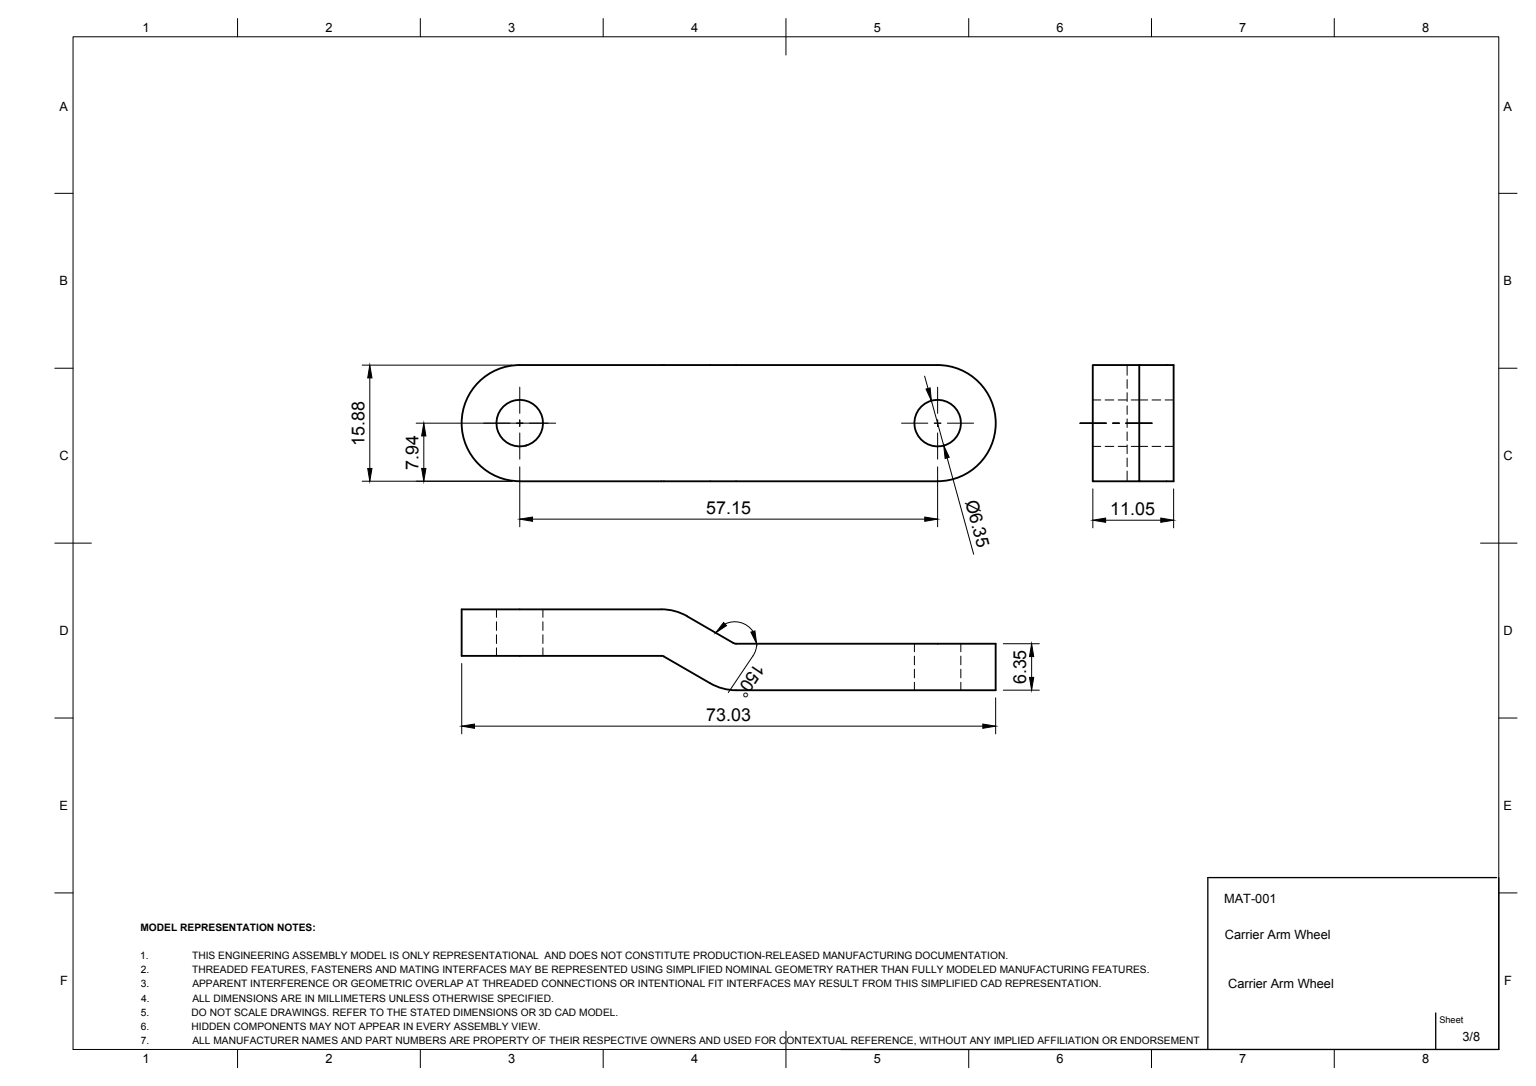
ISO-10303-21;
HEADER;
/* Generated by software containing ST-Developer
 * from STEP Tools, Inc. (www.steptools.com) 
 */

FILE_DESCRIPTION(
/* description */ ('STEP AP214'),
/* implementation_level */ '2;1');

FILE_NAME(
/* name */ 'Carrier Arm Wheel.step',
/* time_stamp */ '2026-11-14T04:30:00-08:00',
/* author */ (''),
/* organization */ (''),
/* preprocessor_version */ 'ST-DEVELOPER v20.2',
/* originating_system */ 'Autodesk Translation Framework v15.17.0.0',
/* authorisation */ '');

FILE_SCHEMA (('AUTOMOTIVE_DESIGN { 1 0 10303 214 3 1 1 }'));
ENDSEC;

DATA;
#10=MECHANICAL_DESIGN_GEOMETRIC_PRESENTATION_REPRESENTATION('',(#129),#40809);
#113=SHAPE_REPRESENTATION_RELATIONSHIP('SRR','None',#40863,#121);
#121=ADVANCED_BREP_SHAPE_REPRESENTATION('',(#137),#40807);
#129=STYLED_ITEM('',(#40906),#137);
#137=MANIFOLD_SOLID_BREP('Body1',#6304);
#313=PLANE('',#7024);
#314=PLANE('',#7025);
#315=PLANE('',#7026);
#316=PLANE('',#7027);
#317=PLANE('',#7031);
#318=PLANE('',#7032);
#319=PLANE('',#7033);
#320=PLANE('',#7034);
#321=PLANE('',#7035);
#322=PLANE('',#7038);
#323=PLANE('',#7043);
#324=PLANE('',#7046);
#325=PLANE('',#7051);
#326=PLANE('',#7052);
#327=PLANE('',#7053);
#328=PLANE('',#7054);
#355=FACE_BOUND('',#1227,.T.);
#356=FACE_BOUND('',#1230,.T.);
#357=FACE_BOUND('',#1241,.T.);
#358=FACE_BOUND('',#1244,.T.);
#815=FACE_OUTER_BOUND('',#1218,.T.);
#816=FACE_OUTER_BOUND('',#1219,.T.);
#817=FACE_OUTER_BOUND('',#1220,.T.);
#818=FACE_OUTER_BOUND('',#1221,.T.);
#819=FACE_OUTER_BOUND('',#1222,.T.);
#820=FACE_OUTER_BOUND('',#1223,.T.);
#821=FACE_OUTER_BOUND('',#1224,.T.);
#822=FACE_OUTER_BOUND('',#1225,.T.);
#823=FACE_OUTER_BOUND('',#1226,.T.);
#824=FACE_OUTER_BOUND('',#1228,.T.);
#825=FACE_OUTER_BOUND('',#1229,.T.);
#826=FACE_OUTER_BOUND('',#1231,.T.);
#827=FACE_OUTER_BOUND('',#1232,.T.);
#828=FACE_OUTER_BOUND('',#1233,.T.);
#829=FACE_OUTER_BOUND('',#1234,.T.);
#830=FACE_OUTER_BOUND('',#1235,.T.);
#831=FACE_OUTER_BOUND('',#1236,.T.);
#832=FACE_OUTER_BOUND('',#1237,.T.);
#833=FACE_OUTER_BOUND('',#1238,.T.);
#834=FACE_OUTER_BOUND('',#1239,.T.);
#835=FACE_OUTER_BOUND('',#1240,.T.);
#836=FACE_OUTER_BOUND('',#1242,.T.);
#837=FACE_OUTER_BOUND('',#1243,.T.);
#838=FACE_OUTER_BOUND('',#1245,.T.);
#1218=EDGE_LOOP('',(#5478,#5479,#5480,#5481));
#1219=EDGE_LOOP('',(#5482,#5483,#5484,#5485));
#1220=EDGE_LOOP('',(#5486,#5487,#5488,#5489));
#1221=EDGE_LOOP('',(#5490,#5491,#5492,#5493));
#1222=EDGE_LOOP('',(#5494,#5495,#5496,#5497));
#1223=EDGE_LOOP('',(#5498,#5499,#5500,#5501));
#1224=EDGE_LOOP('',(#5502,#5503,#5504,#5505));
#1225=EDGE_LOOP('',(#5506,#5507,#5508,#5509));
#1226=EDGE_LOOP('',(#5510,#5511,#5512,#5513));
#1227=EDGE_LOOP('',(#5514));
#1228=EDGE_LOOP('',(#5515,#5516,#5517,#5518));
#1229=EDGE_LOOP('',(#5519,#5520,#5521,#5522));
#1230=EDGE_LOOP('',(#5523));
#1231=EDGE_LOOP('',(#5524,#5525,#5526,#5527));
#1232=EDGE_LOOP('',(#5528,#5529,#5530,#5531));
#1233=EDGE_LOOP('',(#5532,#5533,#5534,#5535));
#1234=EDGE_LOOP('',(#5536,#5537,#5538,#5539));
#1235=EDGE_LOOP('',(#5540,#5541,#5542,#5543));
#1236=EDGE_LOOP('',(#5544,#5545,#5546,#5547));
#1237=EDGE_LOOP('',(#5548,#5549,#5550,#5551));
#1238=EDGE_LOOP('',(#5552,#5553,#5554,#5555));
#1239=EDGE_LOOP('',(#5556,#5557,#5558,#5559));
#1240=EDGE_LOOP('',(#5560,#5561,#5562,#5563));
#1241=EDGE_LOOP('',(#5564));
#1242=EDGE_LOOP('',(#5565,#5566,#5567,#5568));
#1243=EDGE_LOOP('',(#5569,#5570,#5571,#5572));
#1244=EDGE_LOOP('',(#5573));
#1245=EDGE_LOOP('',(#5574,#5575,#5576,#5577));
#1623=CIRCLE('',#7016,3.175);
#1624=CIRCLE('',#7017,3.175);
#1625=CIRCLE('',#7019,7.94000000000001);
#1626=CIRCLE('',#7020,7.94000000000001);
#1627=CIRCLE('',#7022,3.175);
#1628=CIRCLE('',#7023,3.175);
#1629=CIRCLE('',#7029,7.94000000000001);
#1630=CIRCLE('',#7030,7.94000000000001);
#1631=CIRCLE('',#7036,0.7366);
#1632=CIRCLE('',#7037,7.0866);
#1633=CIRCLE('',#7039,0.7366);
#1634=CIRCLE('',#7040,7.0866);
#1635=CIRCLE('',#7044,7.0866);
#1636=CIRCLE('',#7045,0.7366);
#1637=CIRCLE('',#7047,7.0866);
#1638=CIRCLE('',#7048,0.7366);
#2071=LINE('',#40433,#2389);
#2072=LINE('',#40440,#2390);
#2073=LINE('',#40443,#2391);
#2074=LINE('',#40448,#2392);
#2075=LINE('',#40453,#2393);
#2076=LINE('',#40455,#2394);
#2077=LINE('',#40457,#2395);
#2078=LINE('',#40458,#2396);
#2079=LINE('',#40462,#2397);
#2080=LINE('',#40463,#2398);
#2081=LINE('',#40464,#2399);
#2082=LINE('',#40467,#2400);
#2083=LINE('',#40469,#2401);
#2084=LINE('',#40470,#2402);
#2085=LINE('',#40472,#2403);
#2086=LINE('',#40473,#2404);
#2087=LINE('',#40479,#2405);
#2088=LINE('',#40482,#2406);
#2089=LINE('',#40486,#2407);
#2090=LINE('',#40487,#2408);
#2091=LINE('',#40488,#2409);
#2092=LINE('',#40491,#2410);
#2093=LINE('',#40492,#2411);
#2094=LINE('',#40495,#2412);
#2095=LINE('',#40496,#2413);
#2096=LINE('',#40498,#2414);
#2097=LINE('',#40510,#2415);
#2098=LINE('',#40517,#2416);
#2099=LINE('',#40520,#2417);
#2100=LINE('',#40522,#2418);
#2101=LINE('',#40524,#2419);
#2102=LINE('',#40525,#2420);
#2103=LINE('',#40527,#2421);
#2104=LINE('',#40529,#2422);
#2389=VECTOR('',#8673,3.175);
#2390=VECTOR('',#8680,1000.);
#2391=VECTOR('',#8683,1000.);
#2392=VECTOR('',#8688,3.175);
#2393=VECTOR('',#8693,1000.);
#2394=VECTOR('',#8694,1000.);
#2395=VECTOR('',#8695,1000.);
#2396=VECTOR('',#8696,1000.);
#2397=VECTOR('',#8699,1000.);
#2398=VECTOR('',#8700,1000.);
#2399=VECTOR('',#8701,1000.);
#2400=VECTOR('',#8704,1000.);
#2401=VECTOR('',#8705,1000.);
#2402=VECTOR('',#8706,1000.);
#2403=VECTOR('',#8709,1000.);
#2404=VECTOR('',#8710,1000.);
#2405=VECTOR('',#8715,1000.);
#2406=VECTOR('',#8718,1000.);
#2407=VECTOR('',#8721,1000.);
#2408=VECTOR('',#8722,1000.);
#2409=VECTOR('',#8723,1000.);
#2410=VECTOR('',#8726,1000.);
#2411=VECTOR('',#8727,1000.);
#2412=VECTOR('',#8730,1000.);
#2413=VECTOR('',#8731,1000.);
#2414=VECTOR('',#8734,1000.);
#2415=VECTOR('',#8753,1000.);
#2416=VECTOR('',#8762,1000.);
#2417=VECTOR('',#8767,1000.);
#2418=VECTOR('',#8770,1000.);
#2419=VECTOR('',#8773,1000.);
#2420=VECTOR('',#8774,1000.);
#2421=VECTOR('',#8777,1000.);
#2422=VECTOR('',#8780,1000.);
#2935=VERTEX_POINT('',#40430);
#2936=VERTEX_POINT('',#40432);
#2937=VERTEX_POINT('',#40436);
#2938=VERTEX_POINT('',#40437);
#2939=VERTEX_POINT('',#40439);
#2940=VERTEX_POINT('',#40441);
#2941=VERTEX_POINT('',#40445);
#2942=VERTEX_POINT('',#40447);
#2943=VERTEX_POINT('',#40451);
#2944=VERTEX_POINT('',#40452);
#2945=VERTEX_POINT('',#40454);
#2946=VERTEX_POINT('',#40456);
#2947=VERTEX_POINT('',#40460);
#2948=VERTEX_POINT('',#40461);
#2949=VERTEX_POINT('',#40466);
#2950=VERTEX_POINT('',#40468);
#2951=VERTEX_POINT('',#40475);
#2952=VERTEX_POINT('',#40476);
#2953=VERTEX_POINT('',#40478);
#2954=VERTEX_POINT('',#40480);
#2955=VERTEX_POINT('',#40484);
#2956=VERTEX_POINT('',#40485);
#2957=VERTEX_POINT('',#40490);
#2958=VERTEX_POINT('',#40494);
#2959=VERTEX_POINT('',#40508);
#2960=VERTEX_POINT('',#40509);
#2961=VERTEX_POINT('',#40514);
#2962=VERTEX_POINT('',#40516);
#3791=EDGE_CURVE('',#2935,#2935,#1623,.T.);
#3792=EDGE_CURVE('',#2935,#2936,#2071,.T.);
#3793=EDGE_CURVE('',#2936,#2936,#1624,.T.);
#3794=EDGE_CURVE('',#2937,#2938,#1625,.T.);
#3795=EDGE_CURVE('',#2938,#2939,#2072,.T.);
#3796=EDGE_CURVE('',#2940,#2939,#1626,.T.);
#3797=EDGE_CURVE('',#2937,#2940,#2073,.T.);
#3798=EDGE_CURVE('',#2941,#2941,#1627,.T.);
#3799=EDGE_CURVE('',#2941,#2942,#2074,.T.);
#3800=EDGE_CURVE('',#2942,#2942,#1628,.T.);
#3801=EDGE_CURVE('',#2943,#2944,#2075,.T.);
#3802=EDGE_CURVE('',#2944,#2945,#2076,.T.);
#3803=EDGE_CURVE('',#2945,#2946,#2077,.T.);
#3804=EDGE_CURVE('',#2943,#2946,#2078,.T.);
#3805=EDGE_CURVE('',#2947,#2948,#2079,.T.);
#3806=EDGE_CURVE('',#2948,#2944,#2080,.T.);
#3807=EDGE_CURVE('',#2947,#2943,#2081,.T.);
#3808=EDGE_CURVE('',#2945,#2949,#2082,.T.);
#3809=EDGE_CURVE('',#2949,#2950,#2083,.T.);
#3810=EDGE_CURVE('',#2946,#2950,#2084,.T.);
#3811=EDGE_CURVE('',#2948,#2949,#2085,.T.);
#3812=EDGE_CURVE('',#2947,#2950,#2086,.T.);
#3813=EDGE_CURVE('',#2951,#2952,#1629,.T.);
#3814=EDGE_CURVE('',#2953,#2951,#2087,.T.);
#3815=EDGE_CURVE('',#2953,#2954,#1630,.T.);
#3816=EDGE_CURVE('',#2954,#2952,#2088,.T.);
#3817=EDGE_CURVE('',#2955,#2956,#2089,.T.);
#3818=EDGE_CURVE('',#2954,#2955,#2090,.T.);
#3819=EDGE_CURVE('',#2956,#2953,#2091,.T.);
#3820=EDGE_CURVE('',#2955,#2957,#2092,.T.);
#3821=EDGE_CURVE('',#2952,#2957,#2093,.T.);
#3822=EDGE_CURVE('',#2957,#2958,#2094,.T.);
#3823=EDGE_CURVE('',#2958,#2951,#2095,.T.);
#3824=EDGE_CURVE('',#2958,#2956,#2096,.T.);
#3825=EDGE_CURVE('',#2943,#2957,#1631,.T.);
#3826=EDGE_CURVE('',#2947,#2955,#1632,.T.);
#3827=EDGE_CURVE('',#2958,#2946,#1633,.T.);
#3828=EDGE_CURVE('',#2956,#2950,#1634,.T.);
#3829=EDGE_CURVE('',#2959,#2960,#2097,.T.);
#3830=EDGE_CURVE('',#2960,#2944,#1635,.T.);
#3831=EDGE_CURVE('',#2959,#2948,#1636,.T.);
#3832=EDGE_CURVE('',#2945,#2961,#1637,.T.);
#3833=EDGE_CURVE('',#2961,#2962,#2098,.T.);
#3834=EDGE_CURVE('',#2949,#2962,#1638,.T.);
#3835=EDGE_CURVE('',#2959,#2962,#2099,.T.);
#3836=EDGE_CURVE('',#2960,#2961,#2100,.T.);
#3837=EDGE_CURVE('',#2959,#2937,#2101,.T.);
#3838=EDGE_CURVE('',#2938,#2962,#2102,.T.);
#3839=EDGE_CURVE('',#2939,#2961,#2103,.T.);
#3840=EDGE_CURVE('',#2960,#2940,#2104,.T.);
#5478=ORIENTED_EDGE('',*,*,#3791,.F.);
#5479=ORIENTED_EDGE('',*,*,#3792,.T.);
#5480=ORIENTED_EDGE('',*,*,#3793,.T.);
#5481=ORIENTED_EDGE('',*,*,#3792,.F.);
#5482=ORIENTED_EDGE('',*,*,#3794,.T.);
#5483=ORIENTED_EDGE('',*,*,#3795,.T.);
#5484=ORIENTED_EDGE('',*,*,#3796,.F.);
#5485=ORIENTED_EDGE('',*,*,#3797,.F.);
#5486=ORIENTED_EDGE('',*,*,#3798,.F.);
#5487=ORIENTED_EDGE('',*,*,#3799,.T.);
#5488=ORIENTED_EDGE('',*,*,#3800,.T.);
#5489=ORIENTED_EDGE('',*,*,#3799,.F.);
#5490=ORIENTED_EDGE('',*,*,#3801,.T.);
#5491=ORIENTED_EDGE('',*,*,#3802,.T.);
#5492=ORIENTED_EDGE('',*,*,#3803,.T.);
#5493=ORIENTED_EDGE('',*,*,#3804,.F.);
#5494=ORIENTED_EDGE('',*,*,#3805,.T.);
#5495=ORIENTED_EDGE('',*,*,#3806,.T.);
#5496=ORIENTED_EDGE('',*,*,#3801,.F.);
#5497=ORIENTED_EDGE('',*,*,#3807,.F.);
#5498=ORIENTED_EDGE('',*,*,#3803,.F.);
#5499=ORIENTED_EDGE('',*,*,#3808,.T.);
#5500=ORIENTED_EDGE('',*,*,#3809,.T.);
#5501=ORIENTED_EDGE('',*,*,#3810,.F.);
#5502=ORIENTED_EDGE('',*,*,#3811,.F.);
#5503=ORIENTED_EDGE('',*,*,#3805,.F.);
#5504=ORIENTED_EDGE('',*,*,#3812,.T.);
#5505=ORIENTED_EDGE('',*,*,#3809,.F.);
#5506=ORIENTED_EDGE('',*,*,#3813,.F.);
#5507=ORIENTED_EDGE('',*,*,#3814,.F.);
#5508=ORIENTED_EDGE('',*,*,#3815,.T.);
#5509=ORIENTED_EDGE('',*,*,#3816,.T.);
#5510=ORIENTED_EDGE('',*,*,#3817,.F.);
#5511=ORIENTED_EDGE('',*,*,#3818,.F.);
#5512=ORIENTED_EDGE('',*,*,#3815,.F.);
#5513=ORIENTED_EDGE('',*,*,#3819,.F.);
#5514=ORIENTED_EDGE('',*,*,#3798,.T.);
#5515=ORIENTED_EDGE('',*,*,#3818,.T.);
#5516=ORIENTED_EDGE('',*,*,#3820,.T.);
#5517=ORIENTED_EDGE('',*,*,#3821,.F.);
#5518=ORIENTED_EDGE('',*,*,#3816,.F.);
#5519=ORIENTED_EDGE('',*,*,#3821,.T.);
#5520=ORIENTED_EDGE('',*,*,#3822,.T.);
#5521=ORIENTED_EDGE('',*,*,#3823,.T.);
#5522=ORIENTED_EDGE('',*,*,#3813,.T.);
#5523=ORIENTED_EDGE('',*,*,#3800,.F.);
#5524=ORIENTED_EDGE('',*,*,#3823,.F.);
#5525=ORIENTED_EDGE('',*,*,#3824,.T.);
#5526=ORIENTED_EDGE('',*,*,#3819,.T.);
#5527=ORIENTED_EDGE('',*,*,#3814,.T.);
#5528=ORIENTED_EDGE('',*,*,#3807,.T.);
#5529=ORIENTED_EDGE('',*,*,#3825,.T.);
#5530=ORIENTED_EDGE('',*,*,#3820,.F.);
#5531=ORIENTED_EDGE('',*,*,#3826,.F.);
#5532=ORIENTED_EDGE('',*,*,#3824,.F.);
#5533=ORIENTED_EDGE('',*,*,#3827,.T.);
#5534=ORIENTED_EDGE('',*,*,#3810,.T.);
#5535=ORIENTED_EDGE('',*,*,#3828,.F.);
#5536=ORIENTED_EDGE('',*,*,#3828,.T.);
#5537=ORIENTED_EDGE('',*,*,#3812,.F.);
#5538=ORIENTED_EDGE('',*,*,#3826,.T.);
#5539=ORIENTED_EDGE('',*,*,#3817,.T.);
#5540=ORIENTED_EDGE('',*,*,#3827,.F.);
#5541=ORIENTED_EDGE('',*,*,#3822,.F.);
#5542=ORIENTED_EDGE('',*,*,#3825,.F.);
#5543=ORIENTED_EDGE('',*,*,#3804,.T.);
#5544=ORIENTED_EDGE('',*,*,#3829,.T.);
#5545=ORIENTED_EDGE('',*,*,#3830,.T.);
#5546=ORIENTED_EDGE('',*,*,#3806,.F.);
#5547=ORIENTED_EDGE('',*,*,#3831,.F.);
#5548=ORIENTED_EDGE('',*,*,#3808,.F.);
#5549=ORIENTED_EDGE('',*,*,#3832,.T.);
#5550=ORIENTED_EDGE('',*,*,#3833,.T.);
#5551=ORIENTED_EDGE('',*,*,#3834,.F.);
#5552=ORIENTED_EDGE('',*,*,#3834,.T.);
#5553=ORIENTED_EDGE('',*,*,#3835,.F.);
#5554=ORIENTED_EDGE('',*,*,#3831,.T.);
#5555=ORIENTED_EDGE('',*,*,#3811,.T.);
#5556=ORIENTED_EDGE('',*,*,#3832,.F.);
#5557=ORIENTED_EDGE('',*,*,#3802,.F.);
#5558=ORIENTED_EDGE('',*,*,#3830,.F.);
#5559=ORIENTED_EDGE('',*,*,#3836,.T.);
#5560=ORIENTED_EDGE('',*,*,#3837,.F.);
#5561=ORIENTED_EDGE('',*,*,#3835,.T.);
#5562=ORIENTED_EDGE('',*,*,#3838,.F.);
#5563=ORIENTED_EDGE('',*,*,#3794,.F.);
#5564=ORIENTED_EDGE('',*,*,#3791,.T.);
#5565=ORIENTED_EDGE('',*,*,#3833,.F.);
#5566=ORIENTED_EDGE('',*,*,#3839,.F.);
#5567=ORIENTED_EDGE('',*,*,#3795,.F.);
#5568=ORIENTED_EDGE('',*,*,#3838,.T.);
#5569=ORIENTED_EDGE('',*,*,#3836,.F.);
#5570=ORIENTED_EDGE('',*,*,#3840,.T.);
#5571=ORIENTED_EDGE('',*,*,#3796,.T.);
#5572=ORIENTED_EDGE('',*,*,#3839,.T.);
#5573=ORIENTED_EDGE('',*,*,#3793,.F.);
#5574=ORIENTED_EDGE('',*,*,#3829,.F.);
#5575=ORIENTED_EDGE('',*,*,#3837,.T.);
#5576=ORIENTED_EDGE('',*,*,#3797,.T.);
#5577=ORIENTED_EDGE('',*,*,#3840,.F.);
#5889=CYLINDRICAL_SURFACE('',#7015,3.175);
#5890=CYLINDRICAL_SURFACE('',#7018,7.94000000000001);
#5891=CYLINDRICAL_SURFACE('',#7021,3.175);
#5892=CYLINDRICAL_SURFACE('',#7028,7.94000000000001);
#5893=CYLINDRICAL_SURFACE('',#7041,7.0866);
#5894=CYLINDRICAL_SURFACE('',#7042,0.7366);
#5895=CYLINDRICAL_SURFACE('',#7049,0.7366);
#5896=CYLINDRICAL_SURFACE('',#7050,7.0866);
#6230=ADVANCED_FACE('',(#815),#5889,.F.);
#6231=ADVANCED_FACE('',(#816),#5890,.T.);
#6232=ADVANCED_FACE('',(#817),#5891,.F.);
#6233=ADVANCED_FACE('',(#818),#313,.T.);
#6234=ADVANCED_FACE('',(#819),#314,.T.);
#6235=ADVANCED_FACE('',(#820),#315,.T.);
#6236=ADVANCED_FACE('',(#821),#316,.F.);
#6237=ADVANCED_FACE('',(#822),#5892,.T.);
#6238=ADVANCED_FACE('',(#823,#355),#317,.F.);
#6239=ADVANCED_FACE('',(#824),#318,.T.);
#6240=ADVANCED_FACE('',(#825,#356),#319,.T.);
#6241=ADVANCED_FACE('',(#826),#320,.T.);
#6242=ADVANCED_FACE('',(#827),#321,.T.);
#6243=ADVANCED_FACE('',(#828),#322,.T.);
#6244=ADVANCED_FACE('',(#829),#5893,.T.);
#6245=ADVANCED_FACE('',(#830),#5894,.F.);
#6246=ADVANCED_FACE('',(#831),#323,.F.);
#6247=ADVANCED_FACE('',(#832),#324,.F.);
#6248=ADVANCED_FACE('',(#833),#5895,.F.);
#6249=ADVANCED_FACE('',(#834),#5896,.T.);
#6250=ADVANCED_FACE('',(#835,#357),#325,.F.);
#6251=ADVANCED_FACE('',(#836),#326,.T.);
#6252=ADVANCED_FACE('',(#837,#358),#327,.T.);
#6253=ADVANCED_FACE('',(#838),#328,.T.);
#6304=CLOSED_SHELL('',(#6230,#6231,#6232,#6233,#6234,#6235,#6236,#6237,
#6238,#6239,#6240,#6241,#6242,#6243,#6244,#6245,#6246,#6247,#6248,#6249,
#6250,#6251,#6252,#6253));
#7014=AXIS2_PLACEMENT_3D('',#40428,#8667,#8668);
#7015=AXIS2_PLACEMENT_3D('',#40429,#8669,#8670);
#7016=AXIS2_PLACEMENT_3D('',#40431,#8671,#8672);
#7017=AXIS2_PLACEMENT_3D('',#40434,#8674,#8675);
#7018=AXIS2_PLACEMENT_3D('',#40435,#8676,#8677);
#7019=AXIS2_PLACEMENT_3D('',#40438,#8678,#8679);
#7020=AXIS2_PLACEMENT_3D('',#40442,#8681,#8682);
#7021=AXIS2_PLACEMENT_3D('',#40444,#8684,#8685);
#7022=AXIS2_PLACEMENT_3D('',#40446,#8686,#8687);
#7023=AXIS2_PLACEMENT_3D('',#40449,#8689,#8690);
#7024=AXIS2_PLACEMENT_3D('',#40450,#8691,#8692);
#7025=AXIS2_PLACEMENT_3D('',#40459,#8697,#8698);
#7026=AXIS2_PLACEMENT_3D('',#40465,#8702,#8703);
#7027=AXIS2_PLACEMENT_3D('',#40471,#8707,#8708);
#7028=AXIS2_PLACEMENT_3D('',#40474,#8711,#8712);
#7029=AXIS2_PLACEMENT_3D('',#40477,#8713,#8714);
#7030=AXIS2_PLACEMENT_3D('',#40481,#8716,#8717);
#7031=AXIS2_PLACEMENT_3D('',#40483,#8719,#8720);
#7032=AXIS2_PLACEMENT_3D('',#40489,#8724,#8725);
#7033=AXIS2_PLACEMENT_3D('',#40493,#8728,#8729);
#7034=AXIS2_PLACEMENT_3D('',#40497,#8732,#8733);
#7035=AXIS2_PLACEMENT_3D('',#40499,#8735,#8736);
#7036=AXIS2_PLACEMENT_3D('',#40500,#8737,#8738);
#7037=AXIS2_PLACEMENT_3D('',#40501,#8739,#8740);
#7038=AXIS2_PLACEMENT_3D('',#40502,#8741,#8742);
#7039=AXIS2_PLACEMENT_3D('',#40503,#8743,#8744);
#7040=AXIS2_PLACEMENT_3D('',#40504,#8745,#8746);
#7041=AXIS2_PLACEMENT_3D('',#40505,#8747,#8748);
#7042=AXIS2_PLACEMENT_3D('',#40506,#8749,#8750);
#7043=AXIS2_PLACEMENT_3D('',#40507,#8751,#8752);
#7044=AXIS2_PLACEMENT_3D('',#40511,#8754,#8755);
#7045=AXIS2_PLACEMENT_3D('',#40512,#8756,#8757);
#7046=AXIS2_PLACEMENT_3D('',#40513,#8758,#8759);
#7047=AXIS2_PLACEMENT_3D('',#40515,#8760,#8761);
#7048=AXIS2_PLACEMENT_3D('',#40518,#8763,#8764);
#7049=AXIS2_PLACEMENT_3D('',#40519,#8765,#8766);
#7050=AXIS2_PLACEMENT_3D('',#40521,#8768,#8769);
#7051=AXIS2_PLACEMENT_3D('',#40523,#8771,#8772);
#7052=AXIS2_PLACEMENT_3D('',#40526,#8775,#8776);
#7053=AXIS2_PLACEMENT_3D('',#40528,#8778,#8779);
#7054=AXIS2_PLACEMENT_3D('',#40530,#8781,#8782);
#8667=DIRECTION('axis',(0.,0.,1.));
#8668=DIRECTION('refdir',(1.,0.,0.));
#8669=DIRECTION('center_axis',(1.,0.,0.));
#8670=DIRECTION('ref_axis',(0.,0.,-1.));
#8671=DIRECTION('center_axis',(1.,0.,0.));
#8672=DIRECTION('ref_axis',(0.,0.,-1.));
#8673=DIRECTION('',(1.,0.,0.));
#8674=DIRECTION('center_axis',(1.,0.,0.));
#8675=DIRECTION('ref_axis',(0.,0.,-1.));
#8676=DIRECTION('center_axis',(1.,0.,0.));
#8677=DIRECTION('ref_axis',(0.,0.,-1.));
#8678=DIRECTION('center_axis',(1.,0.,0.));
#8679=DIRECTION('ref_axis',(0.,0.,-1.));
#8680=DIRECTION('',(1.,0.,0.));
#8681=DIRECTION('center_axis',(1.,0.,0.));
#8682=DIRECTION('ref_axis',(0.,0.,-1.));
#8683=DIRECTION('',(1.,0.,0.));
#8684=DIRECTION('center_axis',(1.,0.,0.));
#8685=DIRECTION('ref_axis',(0.,0.,-1.));
#8686=DIRECTION('center_axis',(1.,0.,0.));
#8687=DIRECTION('ref_axis',(0.,0.,-1.));
#8688=DIRECTION('',(1.,0.,0.));
#8689=DIRECTION('center_axis',(1.,0.,0.));
#8690=DIRECTION('ref_axis',(0.,0.,-1.));
#8691=DIRECTION('center_axis',(0.866025403784438,0.,0.500000000000001));
#8692=DIRECTION('ref_axis',(0.500000000000001,0.,-0.866025403784438));
#8693=DIRECTION('',(0.500000000000001,1.82123199577618E-16,-0.866025403784438));
#8694=DIRECTION('',(0.,1.,0.));
#8695=DIRECTION('',(-0.500000000000001,-1.82123199577618E-16,0.866025403784438));
#8696=DIRECTION('',(0.,1.,0.));
#8697=DIRECTION('center_axis',(9.10615997888089E-17,-1.,-1.5772331745272E-16));
#8698=DIRECTION('ref_axis',(0.500000000000001,1.82123199577618E-16,-0.866025403784438));
#8699=DIRECTION('',(0.500000000000001,1.82123199577618E-16,-0.866025403784438));
#8700=DIRECTION('',(0.866025403784438,1.11518296706602E-32,0.500000000000001));
#8701=DIRECTION('',(0.866025403784438,1.11518296706602E-32,0.500000000000001));
#8702=DIRECTION('center_axis',(-9.10615997888089E-17,1.,1.5772331745272E-16));
#8703=DIRECTION('ref_axis',(-0.500000000000001,-1.82123199577618E-16,0.866025403784438));
#8704=DIRECTION('',(-0.866025403784438,-1.11518296706602E-32,-0.500000000000001));
#8705=DIRECTION('',(-0.500000000000001,-1.82123199577618E-16,0.866025403784438));
#8706=DIRECTION('',(-0.866025403784438,-1.11518296706602E-32,-0.500000000000001));
#8707=DIRECTION('center_axis',(0.866025403784438,0.,0.500000000000001));
#8708=DIRECTION('ref_axis',(0.500000000000001,0.,-0.866025403784438));
#8709=DIRECTION('',(0.,1.,0.));
#8710=DIRECTION('',(0.,1.,0.));
#8711=DIRECTION('center_axis',(1.,0.,0.));
#8712=DIRECTION('ref_axis',(0.,1.22464679914735E-16,1.));
#8713=DIRECTION('center_axis',(1.,0.,0.));
#8714=DIRECTION('ref_axis',(0.,0.,-1.));
#8715=DIRECTION('',(1.,0.,0.));
#8716=DIRECTION('center_axis',(1.,0.,0.));
#8717=DIRECTION('ref_axis',(0.,0.,-1.));
#8718=DIRECTION('',(1.,0.,0.));
#8719=DIRECTION('center_axis',(1.,0.,0.));
#8720=DIRECTION('ref_axis',(0.,0.,-1.));
#8721=DIRECTION('',(0.,1.,0.));
#8722=DIRECTION('',(0.,1.82123199577618E-16,-1.));
#8723=DIRECTION('',(0.,-1.82123199577618E-16,1.));
#8724=DIRECTION('center_axis',(0.,-1.,-1.82123199577617E-16));
#8725=DIRECTION('ref_axis',(0.,1.82123199577618E-16,-1.));
#8726=DIRECTION('',(1.,1.11518296706602E-32,-6.12323399573677E-17));
#8727=DIRECTION('',(0.,1.82123199577618E-16,-1.));
#8728=DIRECTION('center_axis',(1.,0.,0.));
#8729=DIRECTION('ref_axis',(0.,0.,-1.));
#8730=DIRECTION('',(0.,1.,0.));
#8731=DIRECTION('',(0.,-1.82123199577618E-16,1.));
#8732=DIRECTION('center_axis',(0.,1.,1.82123199577617E-16));
#8733=DIRECTION('ref_axis',(0.,-1.82123199577618E-16,1.));
#8734=DIRECTION('',(-1.,-1.11518296706602E-32,6.12323399573677E-17));
#8735=DIRECTION('center_axis',(0.,-1.,0.));
#8736=DIRECTION('ref_axis',(0.,0.,-1.));
#8737=DIRECTION('center_axis',(0.,1.,0.));
#8738=DIRECTION('ref_axis',(0.,0.,-1.));
#8739=DIRECTION('center_axis',(0.,1.,0.));
#8740=DIRECTION('ref_axis',(0.,0.,-1.));
#8741=DIRECTION('center_axis',(0.,1.,0.));
#8742=DIRECTION('ref_axis',(0.,0.,1.));
#8743=DIRECTION('center_axis',(0.,-1.,0.));
#8744=DIRECTION('ref_axis',(0.,0.,-1.));
#8745=DIRECTION('center_axis',(0.,-1.,0.));
#8746=DIRECTION('ref_axis',(0.,0.,1.));
#8747=DIRECTION('center_axis',(0.,-1.,0.));
#8748=DIRECTION('ref_axis',(0.,0.,-1.));
#8749=DIRECTION('center_axis',(0.,-1.,0.));
#8750=DIRECTION('ref_axis',(0.,0.,-1.));
#8751=DIRECTION('center_axis',(0.,1.,0.));
#8752=DIRECTION('ref_axis',(0.,0.,1.));
#8753=DIRECTION('',(1.,1.11518296706602E-32,0.));
#8754=DIRECTION('center_axis',(0.,-1.,0.));
#8755=DIRECTION('ref_axis',(0.,0.,-1.));
#8756=DIRECTION('center_axis',(0.,-1.,0.));
#8757=DIRECTION('ref_axis',(0.,0.,1.));
#8758=DIRECTION('center_axis',(0.,-1.,0.));
#8759=DIRECTION('ref_axis',(0.,0.,-1.));
#8760=DIRECTION('center_axis',(0.,1.,0.));
#8761=DIRECTION('ref_axis',(-3.54944407778959E-15,0.,-1.));
#8762=DIRECTION('',(-1.,-1.11518296706602E-32,0.));
#8763=DIRECTION('center_axis',(0.,1.,0.));
#8764=DIRECTION('ref_axis',(0.,0.,-1.));
#8765=DIRECTION('center_axis',(0.,-1.,0.));
#8766=DIRECTION('ref_axis',(0.,0.,-1.));
#8767=DIRECTION('',(0.,1.,0.));
#8768=DIRECTION('center_axis',(0.,-1.,0.));
#8769=DIRECTION('ref_axis',(0.,0.,-1.));
#8770=DIRECTION('',(0.,1.,0.));
#8771=DIRECTION('center_axis',(1.,0.,0.));
#8772=DIRECTION('ref_axis',(0.,0.,-1.));
#8773=DIRECTION('',(0.,1.82123199577618E-16,-1.));
#8774=DIRECTION('',(0.,-1.82123199577618E-16,1.));
#8775=DIRECTION('center_axis',(0.,1.,1.82123199577617E-16));
#8776=DIRECTION('ref_axis',(0.,-1.82123199577618E-16,1.));
#8777=DIRECTION('',(0.,-1.82123199577618E-16,1.));
#8778=DIRECTION('center_axis',(1.,0.,0.));
#8779=DIRECTION('ref_axis',(0.,0.,-1.));
#8780=DIRECTION('',(0.,1.82123199577618E-16,-1.));
#8781=DIRECTION('center_axis',(0.,-1.,-1.82123199577617E-16));
#8782=DIRECTION('ref_axis',(0.,1.82123199577618E-16,-1.));
#40428=CARTESIAN_POINT('',(0.,0.,0.));
#40429=CARTESIAN_POINT('Origin',(-1.64999999999999,1.04982846856907E-14,
-28.575));
#40430=CARTESIAN_POINT('',(-1.64999999999999,1.01094593269614E-14,-25.4));
#40431=CARTESIAN_POINT('Origin',(-1.64999999999999,1.04982846856907E-14,
-28.575));
#40432=CARTESIAN_POINT('',(4.70000000000001,1.01094593269614E-14,-25.4));
#40433=CARTESIAN_POINT('',(-1.64999999999999,1.01094593269614E-14,-25.4));
#40434=CARTESIAN_POINT('Origin',(4.70000000000001,1.04982846856907E-14,
-28.575));
#40435=CARTESIAN_POINT('Origin',(-1.64999999999999,1.04982846856907E-14,
-28.575));
#40436=CARTESIAN_POINT('',(-1.64999999999999,-7.94,-28.575));
#40437=CARTESIAN_POINT('',(-1.64999999999999,7.94000000000002,-28.575));
#40438=CARTESIAN_POINT('Origin',(-1.64999999999999,1.04982846856907E-14,
-28.575));
#40439=CARTESIAN_POINT('',(4.70000000000001,7.94000000000002,-28.575));
#40440=CARTESIAN_POINT('',(-1.64999999999999,7.94000000000002,-28.575));
#40441=CARTESIAN_POINT('',(4.70000000000001,-7.94,-28.575));
#40442=CARTESIAN_POINT('Origin',(4.70000000000001,1.04982846856907E-14,
-28.575));
#40443=CARTESIAN_POINT('',(-1.64999999999999,-7.94,-28.575));
#40444=CARTESIAN_POINT('Origin',(-6.35,0.,28.575));
#40445=CARTESIAN_POINT('',(-6.35,-3.88825358729285E-16,31.75));
#40446=CARTESIAN_POINT('Origin',(-6.35,0.,28.575));
#40447=CARTESIAN_POINT('',(0.,-3.88825358729285E-16,31.75));
#40448=CARTESIAN_POINT('',(-6.35,-3.88825358729285E-16,31.75));
#40449=CARTESIAN_POINT('Origin',(0.,0.,28.575));
#40450=CARTESIAN_POINT('Origin',(-14.7008415550852,0.,26.2892875975978));
#40451=CARTESIAN_POINT('',(0.0986856875723831,-7.94000000000001,0.655754485315154));
#40452=CARTESIAN_POINT('',(3.75057562645881,-7.94,-5.66950443248573));
#40453=CARTESIAN_POINT('',(-14.7008415550852,-7.94000000000001,26.2892875975978));
#40454=CARTESIAN_POINT('',(3.75057562645882,7.94000000000002,-5.66950443248573));
#40455=CARTESIAN_POINT('',(3.75057562645881,0.,-5.66950443248573));
#40456=CARTESIAN_POINT('',(0.0986856875723831,7.94000000000002,0.655754485315154));
#40457=CARTESIAN_POINT('',(-14.7008415550852,7.94000000000001,26.2892875975978));
#40458=CARTESIAN_POINT('',(0.0986856875723831,0.,0.655754485315154));
#40459=CARTESIAN_POINT('Origin',(-20.2001028691164,-7.94000000000001,23.1142875975978));
#40460=CARTESIAN_POINT('',(-5.4005756264588,-7.94000000000001,-2.51924551468485));
#40461=CARTESIAN_POINT('',(-1.74868568757237,-7.94000000000001,-8.84450443248573));
#40462=CARTESIAN_POINT('',(-20.2001028691164,-7.94000000000001,23.1142875975978));
#40463=CARTESIAN_POINT('',(-1.74868568757237,-7.94,-8.84450443248573));
#40464=CARTESIAN_POINT('',(-5.4005756264588,-7.94000000000001,-2.51924551468485));
#40465=CARTESIAN_POINT('Origin',(-20.2001028691164,7.94000000000001,23.1142875975978));
#40466=CARTESIAN_POINT('',(-1.74868568757237,7.94000000000002,-8.84450443248573));
#40467=CARTESIAN_POINT('',(-1.74868568757237,7.94000000000002,-8.84450443248573));
#40468=CARTESIAN_POINT('',(-5.4005756264588,7.94000000000002,-2.51924551468485));
#40469=CARTESIAN_POINT('',(-20.2001028691164,7.94000000000001,23.1142875975978));
#40470=CARTESIAN_POINT('',(-5.4005756264588,7.94000000000002,-2.51924551468485));
#40471=CARTESIAN_POINT('Origin',(-20.2001028691164,0.,23.1142875975978));
#40472=CARTESIAN_POINT('',(-1.74868568757237,0.,-8.84450443248573));
#40473=CARTESIAN_POINT('',(-5.4005756264588,0.,-2.51924551468485));
#40474=CARTESIAN_POINT('Origin',(-6.35,0.,28.575));
#40475=CARTESIAN_POINT('',(0.,7.94000000000001,28.575));
#40476=CARTESIAN_POINT('',(0.,-7.94000000000001,28.575));
#40477=CARTESIAN_POINT('Origin',(0.,0.,28.575));
#40478=CARTESIAN_POINT('',(-6.35,7.94000000000001,28.575));
#40479=CARTESIAN_POINT('',(-6.35,7.94000000000001,28.575));
#40480=CARTESIAN_POINT('',(-6.35,-7.94000000000001,28.575));
#40481=CARTESIAN_POINT('Origin',(-6.35,0.,28.575));
#40482=CARTESIAN_POINT('',(-6.35,-7.94000000000001,28.575));
#40483=CARTESIAN_POINT('Origin',(-6.35,0.,28.575));
#40484=CARTESIAN_POINT('',(-6.35,-7.94000000000001,1.02405448531516));
#40485=CARTESIAN_POINT('',(-6.35,7.94000000000002,1.02405448531516));
#40486=CARTESIAN_POINT('',(-6.35,0.,1.02405448531516));
#40487=CARTESIAN_POINT('',(-6.35,-7.94000000000001,28.575));
#40488=CARTESIAN_POINT('',(-6.35,7.94000000000001,28.575));
#40489=CARTESIAN_POINT('Origin',(-6.35,-7.94000000000001,28.575));
#40490=CARTESIAN_POINT('',(0.,-7.94000000000001,1.02405448531516));
#40491=CARTESIAN_POINT('',(-6.35,-7.94000000000001,1.02405448531516));
#40492=CARTESIAN_POINT('',(0.,-7.94000000000001,28.575));
#40493=CARTESIAN_POINT('Origin',(0.,0.,28.575));
#40494=CARTESIAN_POINT('',(0.,7.94000000000002,1.02405448531516));
#40495=CARTESIAN_POINT('',(0.,0.,1.02405448531516));
#40496=CARTESIAN_POINT('',(0.,7.94000000000001,28.575));
#40497=CARTESIAN_POINT('Origin',(-6.35,7.94000000000001,28.575));
#40498=CARTESIAN_POINT('',(-6.35,7.94000000000002,1.02405448531516));
#40499=CARTESIAN_POINT('Origin',(0.7366,-7.94000000000001,1.02405448531516));
#40500=CARTESIAN_POINT('Origin',(0.7366,-7.94000000000001,1.02405448531516));
#40501=CARTESIAN_POINT('Origin',(0.7366,-7.94000000000001,1.02405448531516));
#40502=CARTESIAN_POINT('Origin',(0.7366,7.94000000000002,1.02405448531516));
#40503=CARTESIAN_POINT('Origin',(0.7366,7.94000000000002,1.02405448531516));
#40504=CARTESIAN_POINT('Origin',(0.7366,7.94000000000002,1.02405448531516));
#40505=CARTESIAN_POINT('Origin',(0.7366,17.2247394858551,1.02405448531516));
#40506=CARTESIAN_POINT('Origin',(0.7366,17.2247394858551,1.02405448531516));
#40507=CARTESIAN_POINT('Origin',(-2.38659999999999,-7.94000000000001,-9.21280443248573));
#40508=CARTESIAN_POINT('',(-1.64999999999998,-7.94,-9.21280443248573));
#40509=CARTESIAN_POINT('',(4.70000000000002,-7.94,-9.21280443248573));
#40510=CARTESIAN_POINT('',(-1.64999999999999,-7.94,-9.21280443248573));
#40511=CARTESIAN_POINT('Origin',(-2.38659999999999,-7.94000000000001,-9.21280443248573));
#40512=CARTESIAN_POINT('Origin',(-2.38659999999999,-7.94000000000001,-9.21280443248573));
#40513=CARTESIAN_POINT('Origin',(-2.38659999999999,7.94000000000002,-9.21280443248573));
#40514=CARTESIAN_POINT('',(4.70000000000002,7.94000000000002,-9.21280443248573));
#40515=CARTESIAN_POINT('Origin',(-2.38659999999999,7.94000000000002,-9.21280443248573));
#40516=CARTESIAN_POINT('',(-1.64999999999999,7.94000000000002,-9.21280443248573));
#40517=CARTESIAN_POINT('',(-1.64999999999999,7.94000000000002,-9.21280443248573));
#40518=CARTESIAN_POINT('Origin',(-2.38659999999999,7.94000000000002,-9.21280443248573));
#40519=CARTESIAN_POINT('Origin',(-2.38659999999999,17.8666679381969,-9.21280443248573));
#40520=CARTESIAN_POINT('',(-1.64999999999998,0.,-9.21280443248573));
#40521=CARTESIAN_POINT('Origin',(-2.38659999999999,17.8666679381969,-9.21280443248573));
#40522=CARTESIAN_POINT('',(4.70000000000002,0.,-9.21280443248573));
#40523=CARTESIAN_POINT('Origin',(-1.64999999999999,0.,29.7381389012326));
#40524=CARTESIAN_POINT('',(-1.64999999999998,-7.94000000000001,29.7381389012326));
#40525=CARTESIAN_POINT('',(-1.64999999999998,7.94000000000001,29.7381389012326));
#40526=CARTESIAN_POINT('Origin',(-1.64999999999998,7.94000000000001,29.7381389012326));
#40527=CARTESIAN_POINT('',(4.70000000000002,7.94000000000001,29.7381389012326));
#40528=CARTESIAN_POINT('Origin',(4.70000000000002,0.,29.7381389012326));
#40529=CARTESIAN_POINT('',(4.70000000000002,-7.94000000000001,29.7381389012326));
#40530=CARTESIAN_POINT('Origin',(-1.64999999999998,-7.94000000000001,29.7381389012326));
#40797=UNCERTAINTY_MEASURE_WITH_UNIT(LENGTH_MEASURE(0.01),#40810,
'DISTANCE_ACCURACY_VALUE',
'Maximum model space distance between geometric entities at asserted c
onnectivities');
#40799=UNCERTAINTY_MEASURE_WITH_UNIT(LENGTH_MEASURE(0.01),#40810,
'DISTANCE_ACCURACY_VALUE',
'Maximum model space distance between geometric entities at asserted c
onnectivities');
#40807=(
GEOMETRIC_REPRESENTATION_CONTEXT(3)
GLOBAL_UNCERTAINTY_ASSIGNED_CONTEXT((#40797))
GLOBAL_UNIT_ASSIGNED_CONTEXT((#40810,#40812,#40813))
REPRESENTATION_CONTEXT('','3D')
);
#40809=(
GEOMETRIC_REPRESENTATION_CONTEXT(3)
GLOBAL_UNCERTAINTY_ASSIGNED_CONTEXT((#40799))
GLOBAL_UNIT_ASSIGNED_CONTEXT((#40810,#40812,#40813))
REPRESENTATION_CONTEXT('','3D')
);
#40810=(
LENGTH_UNIT()
NAMED_UNIT(*)
SI_UNIT(.MILLI.,.METRE.)
);
#40812=(
NAMED_UNIT(*)
PLANE_ANGLE_UNIT()
SI_UNIT($,.RADIAN.)
);
#40813=(
NAMED_UNIT(*)
SI_UNIT($,.STERADIAN.)
SOLID_ANGLE_UNIT()
);
#40821=SHAPE_DEFINITION_REPRESENTATION(#40830,#40863);
#40830=PRODUCT_DEFINITION_SHAPE('',$,#40873);
#40863=SHAPE_REPRESENTATION('',(#7014),#40807);
#40865=PRODUCT_DEFINITION_CONTEXT('part definition',#40894,'design');
#40873=PRODUCT_DEFINITION('Carrier Arm Wheel','Carrier Arm Wheel',#40882,
#40865);
#40882=PRODUCT_DEFINITION_FORMATION('',$,#40903);
#40894=APPLICATION_CONTEXT(
'Core Data for Automotive Mechanical Design Process');
#40895=PRODUCT_CONTEXT('part definition',#40894,'mechanical');
#40903=PRODUCT('Carrier Arm Wheel','Carrier Arm Wheel',$,(#40895));
#40906=PRESENTATION_STYLE_ASSIGNMENT((#40911));
#40911=SURFACE_STYLE_USAGE(.BOTH.,#40916);
#40916=SURFACE_SIDE_STYLE('',(#40921));
#40921=SURFACE_STYLE_FILL_AREA(#40926);
#40926=FILL_AREA_STYLE('Opaque(227,224,212)',(#40931));
#40931=FILL_AREA_STYLE_COLOUR('Opaque(227,224,212)',#40936);
#40936=COLOUR_RGB('Opaque(227,224,212)',0.890196078431372,0.87843137254902,
0.831372549019608);
ENDSEC;
END-ISO-10303-21;
